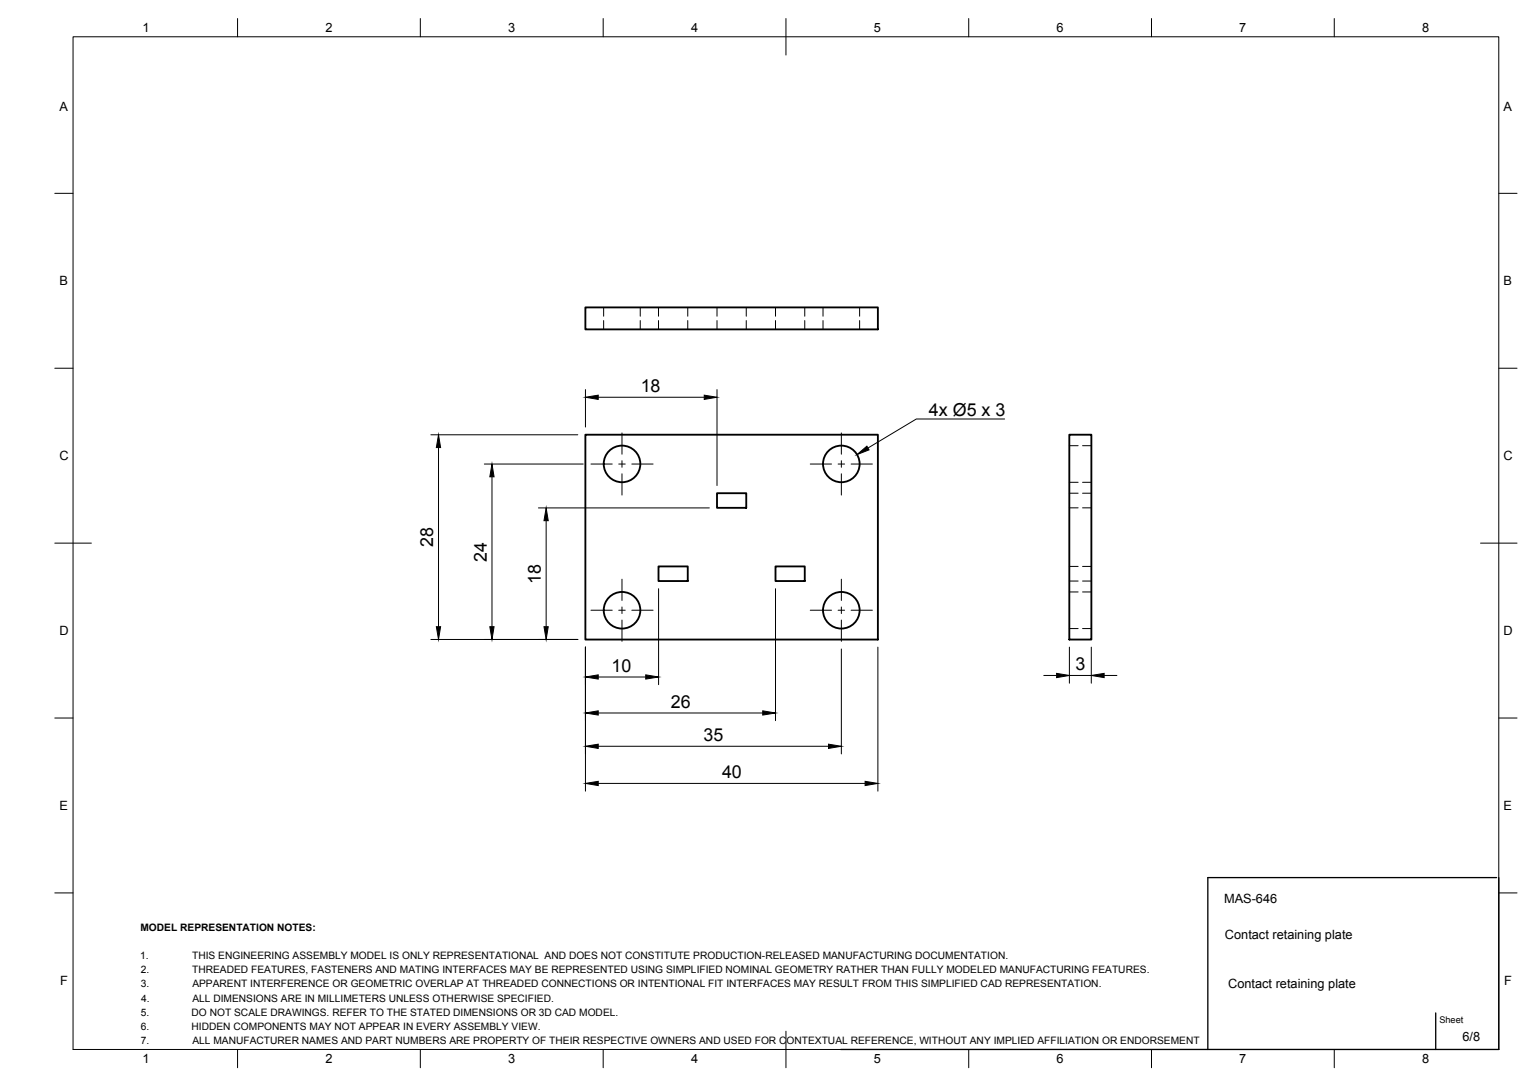
ISO-10303-21;
HEADER;
/* Generated by software containing ST-Developer
 * from STEP Tools, Inc. (www.steptools.com) 
 */

FILE_DESCRIPTION(
/* description */ ('Independent keyed three-contact power inlet for the IEC-connector des
ign category. Longer ground blade, retained contacts, wire termination
 holes and sealed bolted panel interface. Nominal custom interface; IE
C dimensional compatibility and electrical ratings are not assigned.'),

/* implementation_level */ '2;1');

FILE_NAME(
/* name */ 'Contact retaining plate.step',
/* time_stamp */ '2026-11-08T19:55:04-08:00',
/* author */ (''),
/* organization */ (''),
/* preprocessor_version */ 'ST-DEVELOPER v20.2',
/* originating_system */ 'Autodesk Translation Framework v15.17.0.0',
/* authorisation */ '');

FILE_SCHEMA (('AUTOMOTIVE_DESIGN { 1 0 10303 214 3 1 1 }'));
ENDSEC;

DATA;
#10=MECHANICAL_DESIGN_GEOMETRIC_PRESENTATION_REPRESENTATION('',(#112),#21880);
#92=SHAPE_REPRESENTATION_RELATIONSHIP('SRR','None',#21928,#102);
#102=ADVANCED_BREP_SHAPE_REPRESENTATION('',(#122),#21873);
#112=STYLED_ITEM('',(#21987),#122);
#122=MANIFOLD_SOLID_BREP('Body1',#6384);
#171=FACE_BOUND('',#918,.T.);
#172=FACE_BOUND('',#919,.T.);
#173=FACE_BOUND('',#920,.T.);
#174=FACE_BOUND('',#921,.T.);
#175=FACE_BOUND('',#922,.T.);
#176=FACE_BOUND('',#923,.T.);
#177=FACE_BOUND('',#924,.T.);
#178=FACE_BOUND('',#926,.T.);
#179=FACE_BOUND('',#927,.T.);
#180=FACE_BOUND('',#928,.T.);
#181=FACE_BOUND('',#929,.T.);
#182=FACE_BOUND('',#930,.T.);
#183=FACE_BOUND('',#931,.T.);
#184=FACE_BOUND('',#932,.T.);
#253=PLANE('',#6784);
#254=PLANE('',#6785);
#255=PLANE('',#6786);
#256=PLANE('',#6787);
#257=PLANE('',#6788);
#258=PLANE('',#6789);
#259=PLANE('',#6790);
#260=PLANE('',#6791);
#261=PLANE('',#6792);
#262=PLANE('',#6793);
#263=PLANE('',#6794);
#264=PLANE('',#6795);
#265=PLANE('',#6796);
#266=PLANE('',#6797);
#267=PLANE('',#6798);
#268=PLANE('',#6799);
#269=PLANE('',#6800);
#270=PLANE('',#6801);
#525=FACE_OUTER_BOUND('',#897,.T.);
#526=FACE_OUTER_BOUND('',#898,.T.);
#527=FACE_OUTER_BOUND('',#899,.T.);
#528=FACE_OUTER_BOUND('',#900,.T.);
#529=FACE_OUTER_BOUND('',#901,.T.);
#530=FACE_OUTER_BOUND('',#902,.T.);
#531=FACE_OUTER_BOUND('',#903,.T.);
#532=FACE_OUTER_BOUND('',#904,.T.);
#533=FACE_OUTER_BOUND('',#905,.T.);
#534=FACE_OUTER_BOUND('',#906,.T.);
#535=FACE_OUTER_BOUND('',#907,.T.);
#536=FACE_OUTER_BOUND('',#908,.T.);
#537=FACE_OUTER_BOUND('',#909,.T.);
#538=FACE_OUTER_BOUND('',#910,.T.);
#539=FACE_OUTER_BOUND('',#911,.T.);
#540=FACE_OUTER_BOUND('',#912,.T.);
#541=FACE_OUTER_BOUND('',#913,.T.);
#542=FACE_OUTER_BOUND('',#914,.T.);
#543=FACE_OUTER_BOUND('',#915,.T.);
#544=FACE_OUTER_BOUND('',#916,.T.);
#545=FACE_OUTER_BOUND('',#917,.T.);
#546=FACE_OUTER_BOUND('',#925,.T.);
#897=EDGE_LOOP('',(#5075,#5076,#5077,#5078));
#898=EDGE_LOOP('',(#5079,#5080,#5081,#5082));
#899=EDGE_LOOP('',(#5083,#5084,#5085,#5086));
#900=EDGE_LOOP('',(#5087,#5088,#5089,#5090));
#901=EDGE_LOOP('',(#5091,#5092,#5093,#5094));
#902=EDGE_LOOP('',(#5095,#5096,#5097,#5098));
#903=EDGE_LOOP('',(#5099,#5100,#5101,#5102));
#904=EDGE_LOOP('',(#5103,#5104,#5105,#5106));
#905=EDGE_LOOP('',(#5107,#5108,#5109,#5110));
#906=EDGE_LOOP('',(#5111,#5112,#5113,#5114));
#907=EDGE_LOOP('',(#5115,#5116,#5117,#5118));
#908=EDGE_LOOP('',(#5119,#5120,#5121,#5122));
#909=EDGE_LOOP('',(#5123,#5124,#5125,#5126));
#910=EDGE_LOOP('',(#5127,#5128,#5129,#5130));
#911=EDGE_LOOP('',(#5131,#5132,#5133,#5134));
#912=EDGE_LOOP('',(#5135,#5136,#5137,#5138));
#913=EDGE_LOOP('',(#5139,#5140,#5141,#5142));
#914=EDGE_LOOP('',(#5143,#5144,#5145,#5146));
#915=EDGE_LOOP('',(#5147,#5148,#5149,#5150));
#916=EDGE_LOOP('',(#5151,#5152,#5153,#5154));
#917=EDGE_LOOP('',(#5155,#5156,#5157,#5158));
#918=EDGE_LOOP('',(#5159,#5160,#5161,#5162));
#919=EDGE_LOOP('',(#5163,#5164,#5165,#5166));
#920=EDGE_LOOP('',(#5167,#5168,#5169,#5170));
#921=EDGE_LOOP('',(#5171));
#922=EDGE_LOOP('',(#5172));
#923=EDGE_LOOP('',(#5173));
#924=EDGE_LOOP('',(#5174));
#925=EDGE_LOOP('',(#5175,#5176,#5177,#5178));
#926=EDGE_LOOP('',(#5179,#5180,#5181,#5182));
#927=EDGE_LOOP('',(#5183,#5184,#5185,#5186));
#928=EDGE_LOOP('',(#5187,#5188,#5189,#5190));
#929=EDGE_LOOP('',(#5191));
#930=EDGE_LOOP('',(#5192));
#931=EDGE_LOOP('',(#5193));
#932=EDGE_LOOP('',(#5194));
#1128=CIRCLE('',#6773,2.5);
#1129=CIRCLE('',#6774,2.5);
#1130=CIRCLE('',#6776,2.5);
#1131=CIRCLE('',#6777,2.5);
#1132=CIRCLE('',#6779,2.5);
#1133=CIRCLE('',#6780,2.5);
#1134=CIRCLE('',#6782,2.5);
#1135=CIRCLE('',#6783,2.5);
#1787=LINE('',#16163,#2243);
#1788=LINE('',#16169,#2244);
#1789=LINE('',#16175,#2245);
#1790=LINE('',#16181,#2246);
#1791=LINE('',#16186,#2247);
#1792=LINE('',#16188,#2248);
#1793=LINE('',#16190,#2249);
#1794=LINE('',#16191,#2250);
#1795=LINE('',#16194,#2251);
#1796=LINE('',#16196,#2252);
#1797=LINE('',#16197,#2253);
#1798=LINE('',#16200,#2254);
#1799=LINE('',#16202,#2255);
#1800=LINE('',#16203,#2256);
#1801=LINE('',#16205,#2257);
#1802=LINE('',#16206,#2258);
#1803=LINE('',#16210,#2259);
#1804=LINE('',#16212,#2260);
#1805=LINE('',#16214,#2261);
#1806=LINE('',#16215,#2262);
#1807=LINE('',#16218,#2263);
#1808=LINE('',#16220,#2264);
#1809=LINE('',#16221,#2265);
#1810=LINE('',#16224,#2266);
#1811=LINE('',#16226,#2267);
#1812=LINE('',#16227,#2268);
#1813=LINE('',#16229,#2269);
#1814=LINE('',#16230,#2270);
#1815=LINE('',#16234,#2271);
#1816=LINE('',#16236,#2272);
#1817=LINE('',#16238,#2273);
#1818=LINE('',#16239,#2274);
#1819=LINE('',#16242,#2275);
#1820=LINE('',#16244,#2276);
#1821=LINE('',#16245,#2277);
#1822=LINE('',#16248,#2278);
#1823=LINE('',#16250,#2279);
#1824=LINE('',#16251,#2280);
#1825=LINE('',#16253,#2281);
#1826=LINE('',#16254,#2282);
#1827=LINE('',#16258,#2283);
#1828=LINE('',#16260,#2284);
#1829=LINE('',#16262,#2285);
#1830=LINE('',#16263,#2286);
#1831=LINE('',#16266,#2287);
#1832=LINE('',#16268,#2288);
#1833=LINE('',#16269,#2289);
#1834=LINE('',#16272,#2290);
#1835=LINE('',#16274,#2291);
#1836=LINE('',#16275,#2292);
#1837=LINE('',#16277,#2293);
#1838=LINE('',#16278,#2294);
#2243=VECTOR('',#7769,2.5);
#2244=VECTOR('',#7776,2.5);
#2245=VECTOR('',#7783,2.5);
#2246=VECTOR('',#7790,2.5);
#2247=VECTOR('',#7795,10.);
#2248=VECTOR('',#7796,10.);
#2249=VECTOR('',#7797,10.);
#2250=VECTOR('',#7798,10.);
#2251=VECTOR('',#7801,10.);
#2252=VECTOR('',#7802,10.);
#2253=VECTOR('',#7803,10.);
#2254=VECTOR('',#7806,10.);
#2255=VECTOR('',#7807,10.);
#2256=VECTOR('',#7808,10.);
#2257=VECTOR('',#7811,10.);
#2258=VECTOR('',#7812,10.);
#2259=VECTOR('',#7815,10.);
#2260=VECTOR('',#7816,10.);
#2261=VECTOR('',#7817,10.);
#2262=VECTOR('',#7818,10.);
#2263=VECTOR('',#7821,10.);
#2264=VECTOR('',#7822,10.);
#2265=VECTOR('',#7823,10.);
#2266=VECTOR('',#7826,10.);
#2267=VECTOR('',#7827,10.);
#2268=VECTOR('',#7828,10.);
#2269=VECTOR('',#7831,10.);
#2270=VECTOR('',#7832,10.);
#2271=VECTOR('',#7835,10.);
#2272=VECTOR('',#7836,10.);
#2273=VECTOR('',#7837,10.);
#2274=VECTOR('',#7838,10.);
#2275=VECTOR('',#7841,10.);
#2276=VECTOR('',#7842,10.);
#2277=VECTOR('',#7843,10.);
#2278=VECTOR('',#7846,10.);
#2279=VECTOR('',#7847,10.);
#2280=VECTOR('',#7848,10.);
#2281=VECTOR('',#7851,10.);
#2282=VECTOR('',#7852,10.);
#2283=VECTOR('',#7855,10.);
#2284=VECTOR('',#7856,10.);
#2285=VECTOR('',#7857,10.);
#2286=VECTOR('',#7858,10.);
#2287=VECTOR('',#7861,10.);
#2288=VECTOR('',#7862,10.);
#2289=VECTOR('',#7863,10.);
#2290=VECTOR('',#7866,10.);
#2291=VECTOR('',#7867,10.);
#2292=VECTOR('',#7868,10.);
#2293=VECTOR('',#7871,10.);
#2294=VECTOR('',#7872,10.);
#2795=VERTEX_POINT('',#16160);
#2796=VERTEX_POINT('',#16162);
#2797=VERTEX_POINT('',#16166);
#2798=VERTEX_POINT('',#16168);
#2799=VERTEX_POINT('',#16172);
#2800=VERTEX_POINT('',#16174);
#2801=VERTEX_POINT('',#16178);
#2802=VERTEX_POINT('',#16180);
#2803=VERTEX_POINT('',#16184);
#2804=VERTEX_POINT('',#16185);
#2805=VERTEX_POINT('',#16187);
#2806=VERTEX_POINT('',#16189);
#2807=VERTEX_POINT('',#16193);
#2808=VERTEX_POINT('',#16195);
#2809=VERTEX_POINT('',#16199);
#2810=VERTEX_POINT('',#16201);
#2811=VERTEX_POINT('',#16208);
#2812=VERTEX_POINT('',#16209);
#2813=VERTEX_POINT('',#16211);
#2814=VERTEX_POINT('',#16213);
#2815=VERTEX_POINT('',#16217);
#2816=VERTEX_POINT('',#16219);
#2817=VERTEX_POINT('',#16223);
#2818=VERTEX_POINT('',#16225);
#2819=VERTEX_POINT('',#16232);
#2820=VERTEX_POINT('',#16233);
#2821=VERTEX_POINT('',#16235);
#2822=VERTEX_POINT('',#16237);
#2823=VERTEX_POINT('',#16241);
#2824=VERTEX_POINT('',#16243);
#2825=VERTEX_POINT('',#16247);
#2826=VERTEX_POINT('',#16249);
#2827=VERTEX_POINT('',#16256);
#2828=VERTEX_POINT('',#16257);
#2829=VERTEX_POINT('',#16259);
#2830=VERTEX_POINT('',#16261);
#2831=VERTEX_POINT('',#16265);
#2832=VERTEX_POINT('',#16267);
#2833=VERTEX_POINT('',#16271);
#2834=VERTEX_POINT('',#16273);
#3597=EDGE_CURVE('',#2795,#2795,#1128,.T.);
#3598=EDGE_CURVE('',#2795,#2796,#1787,.T.);
#3599=EDGE_CURVE('',#2796,#2796,#1129,.T.);
#3600=EDGE_CURVE('',#2797,#2797,#1130,.T.);
#3601=EDGE_CURVE('',#2797,#2798,#1788,.T.);
#3602=EDGE_CURVE('',#2798,#2798,#1131,.T.);
#3603=EDGE_CURVE('',#2799,#2799,#1132,.T.);
#3604=EDGE_CURVE('',#2799,#2800,#1789,.T.);
#3605=EDGE_CURVE('',#2800,#2800,#1133,.T.);
#3606=EDGE_CURVE('',#2801,#2801,#1134,.T.);
#3607=EDGE_CURVE('',#2801,#2802,#1790,.T.);
#3608=EDGE_CURVE('',#2802,#2802,#1135,.T.);
#3609=EDGE_CURVE('',#2803,#2804,#1791,.T.);
#3610=EDGE_CURVE('',#2803,#2805,#1792,.T.);
#3611=EDGE_CURVE('',#2806,#2805,#1793,.T.);
#3612=EDGE_CURVE('',#2804,#2806,#1794,.T.);
#3613=EDGE_CURVE('',#2807,#2803,#1795,.T.);
#3614=EDGE_CURVE('',#2807,#2808,#1796,.T.);
#3615=EDGE_CURVE('',#2805,#2808,#1797,.T.);
#3616=EDGE_CURVE('',#2809,#2807,#1798,.T.);
#3617=EDGE_CURVE('',#2809,#2810,#1799,.T.);
#3618=EDGE_CURVE('',#2808,#2810,#1800,.T.);
#3619=EDGE_CURVE('',#2804,#2809,#1801,.T.);
#3620=EDGE_CURVE('',#2810,#2806,#1802,.T.);
#3621=EDGE_CURVE('',#2811,#2812,#1803,.T.);
#3622=EDGE_CURVE('',#2811,#2813,#1804,.T.);
#3623=EDGE_CURVE('',#2814,#2813,#1805,.T.);
#3624=EDGE_CURVE('',#2812,#2814,#1806,.T.);
#3625=EDGE_CURVE('',#2815,#2811,#1807,.T.);
#3626=EDGE_CURVE('',#2815,#2816,#1808,.T.);
#3627=EDGE_CURVE('',#2813,#2816,#1809,.T.);
#3628=EDGE_CURVE('',#2817,#2815,#1810,.T.);
#3629=EDGE_CURVE('',#2817,#2818,#1811,.T.);
#3630=EDGE_CURVE('',#2816,#2818,#1812,.T.);
#3631=EDGE_CURVE('',#2812,#2817,#1813,.T.);
#3632=EDGE_CURVE('',#2818,#2814,#1814,.T.);
#3633=EDGE_CURVE('',#2819,#2820,#1815,.T.);
#3634=EDGE_CURVE('',#2819,#2821,#1816,.T.);
#3635=EDGE_CURVE('',#2822,#2821,#1817,.T.);
#3636=EDGE_CURVE('',#2820,#2822,#1818,.T.);
#3637=EDGE_CURVE('',#2823,#2819,#1819,.T.);
#3638=EDGE_CURVE('',#2823,#2824,#1820,.T.);
#3639=EDGE_CURVE('',#2821,#2824,#1821,.T.);
#3640=EDGE_CURVE('',#2825,#2823,#1822,.T.);
#3641=EDGE_CURVE('',#2825,#2826,#1823,.T.);
#3642=EDGE_CURVE('',#2824,#2826,#1824,.T.);
#3643=EDGE_CURVE('',#2820,#2825,#1825,.T.);
#3644=EDGE_CURVE('',#2826,#2822,#1826,.T.);
#3645=EDGE_CURVE('',#2827,#2828,#1827,.T.);
#3646=EDGE_CURVE('',#2828,#2829,#1828,.T.);
#3647=EDGE_CURVE('',#2830,#2829,#1829,.T.);
#3648=EDGE_CURVE('',#2827,#2830,#1830,.T.);
#3649=EDGE_CURVE('',#2831,#2827,#1831,.T.);
#3650=EDGE_CURVE('',#2832,#2830,#1832,.T.);
#3651=EDGE_CURVE('',#2831,#2832,#1833,.T.);
#3652=EDGE_CURVE('',#2833,#2831,#1834,.T.);
#3653=EDGE_CURVE('',#2834,#2832,#1835,.T.);
#3654=EDGE_CURVE('',#2833,#2834,#1836,.T.);
#3655=EDGE_CURVE('',#2828,#2833,#1837,.T.);
#3656=EDGE_CURVE('',#2829,#2834,#1838,.T.);
#5075=ORIENTED_EDGE('',*,*,#3597,.F.);
#5076=ORIENTED_EDGE('',*,*,#3598,.T.);
#5077=ORIENTED_EDGE('',*,*,#3599,.F.);
#5078=ORIENTED_EDGE('',*,*,#3598,.F.);
#5079=ORIENTED_EDGE('',*,*,#3600,.F.);
#5080=ORIENTED_EDGE('',*,*,#3601,.T.);
#5081=ORIENTED_EDGE('',*,*,#3602,.F.);
#5082=ORIENTED_EDGE('',*,*,#3601,.F.);
#5083=ORIENTED_EDGE('',*,*,#3603,.F.);
#5084=ORIENTED_EDGE('',*,*,#3604,.T.);
#5085=ORIENTED_EDGE('',*,*,#3605,.F.);
#5086=ORIENTED_EDGE('',*,*,#3604,.F.);
#5087=ORIENTED_EDGE('',*,*,#3606,.F.);
#5088=ORIENTED_EDGE('',*,*,#3607,.T.);
#5089=ORIENTED_EDGE('',*,*,#3608,.F.);
#5090=ORIENTED_EDGE('',*,*,#3607,.F.);
#5091=ORIENTED_EDGE('',*,*,#3609,.F.);
#5092=ORIENTED_EDGE('',*,*,#3610,.T.);
#5093=ORIENTED_EDGE('',*,*,#3611,.F.);
#5094=ORIENTED_EDGE('',*,*,#3612,.F.);
#5095=ORIENTED_EDGE('',*,*,#3613,.F.);
#5096=ORIENTED_EDGE('',*,*,#3614,.T.);
#5097=ORIENTED_EDGE('',*,*,#3615,.F.);
#5098=ORIENTED_EDGE('',*,*,#3610,.F.);
#5099=ORIENTED_EDGE('',*,*,#3616,.F.);
#5100=ORIENTED_EDGE('',*,*,#3617,.T.);
#5101=ORIENTED_EDGE('',*,*,#3618,.F.);
#5102=ORIENTED_EDGE('',*,*,#3614,.F.);
#5103=ORIENTED_EDGE('',*,*,#3619,.F.);
#5104=ORIENTED_EDGE('',*,*,#3612,.T.);
#5105=ORIENTED_EDGE('',*,*,#3620,.F.);
#5106=ORIENTED_EDGE('',*,*,#3617,.F.);
#5107=ORIENTED_EDGE('',*,*,#3621,.F.);
#5108=ORIENTED_EDGE('',*,*,#3622,.T.);
#5109=ORIENTED_EDGE('',*,*,#3623,.F.);
#5110=ORIENTED_EDGE('',*,*,#3624,.F.);
#5111=ORIENTED_EDGE('',*,*,#3625,.F.);
#5112=ORIENTED_EDGE('',*,*,#3626,.T.);
#5113=ORIENTED_EDGE('',*,*,#3627,.F.);
#5114=ORIENTED_EDGE('',*,*,#3622,.F.);
#5115=ORIENTED_EDGE('',*,*,#3628,.F.);
#5116=ORIENTED_EDGE('',*,*,#3629,.T.);
#5117=ORIENTED_EDGE('',*,*,#3630,.F.);
#5118=ORIENTED_EDGE('',*,*,#3626,.F.);
#5119=ORIENTED_EDGE('',*,*,#3631,.F.);
#5120=ORIENTED_EDGE('',*,*,#3624,.T.);
#5121=ORIENTED_EDGE('',*,*,#3632,.F.);
#5122=ORIENTED_EDGE('',*,*,#3629,.F.);
#5123=ORIENTED_EDGE('',*,*,#3633,.F.);
#5124=ORIENTED_EDGE('',*,*,#3634,.T.);
#5125=ORIENTED_EDGE('',*,*,#3635,.F.);
#5126=ORIENTED_EDGE('',*,*,#3636,.F.);
#5127=ORIENTED_EDGE('',*,*,#3637,.F.);
#5128=ORIENTED_EDGE('',*,*,#3638,.T.);
#5129=ORIENTED_EDGE('',*,*,#3639,.F.);
#5130=ORIENTED_EDGE('',*,*,#3634,.F.);
#5131=ORIENTED_EDGE('',*,*,#3640,.F.);
#5132=ORIENTED_EDGE('',*,*,#3641,.T.);
#5133=ORIENTED_EDGE('',*,*,#3642,.F.);
#5134=ORIENTED_EDGE('',*,*,#3638,.F.);
#5135=ORIENTED_EDGE('',*,*,#3643,.F.);
#5136=ORIENTED_EDGE('',*,*,#3636,.T.);
#5137=ORIENTED_EDGE('',*,*,#3644,.F.);
#5138=ORIENTED_EDGE('',*,*,#3641,.F.);
#5139=ORIENTED_EDGE('',*,*,#3645,.T.);
#5140=ORIENTED_EDGE('',*,*,#3646,.T.);
#5141=ORIENTED_EDGE('',*,*,#3647,.F.);
#5142=ORIENTED_EDGE('',*,*,#3648,.F.);
#5143=ORIENTED_EDGE('',*,*,#3649,.T.);
#5144=ORIENTED_EDGE('',*,*,#3648,.T.);
#5145=ORIENTED_EDGE('',*,*,#3650,.F.);
#5146=ORIENTED_EDGE('',*,*,#3651,.F.);
#5147=ORIENTED_EDGE('',*,*,#3652,.T.);
#5148=ORIENTED_EDGE('',*,*,#3651,.T.);
#5149=ORIENTED_EDGE('',*,*,#3653,.F.);
#5150=ORIENTED_EDGE('',*,*,#3654,.F.);
#5151=ORIENTED_EDGE('',*,*,#3655,.T.);
#5152=ORIENTED_EDGE('',*,*,#3654,.T.);
#5153=ORIENTED_EDGE('',*,*,#3656,.F.);
#5154=ORIENTED_EDGE('',*,*,#3646,.F.);
#5155=ORIENTED_EDGE('',*,*,#3656,.T.);
#5156=ORIENTED_EDGE('',*,*,#3653,.T.);
#5157=ORIENTED_EDGE('',*,*,#3650,.T.);
#5158=ORIENTED_EDGE('',*,*,#3647,.T.);
#5159=ORIENTED_EDGE('',*,*,#3633,.T.);
#5160=ORIENTED_EDGE('',*,*,#3643,.T.);
#5161=ORIENTED_EDGE('',*,*,#3640,.T.);
#5162=ORIENTED_EDGE('',*,*,#3637,.T.);
#5163=ORIENTED_EDGE('',*,*,#3621,.T.);
#5164=ORIENTED_EDGE('',*,*,#3631,.T.);
#5165=ORIENTED_EDGE('',*,*,#3628,.T.);
#5166=ORIENTED_EDGE('',*,*,#3625,.T.);
#5167=ORIENTED_EDGE('',*,*,#3609,.T.);
#5168=ORIENTED_EDGE('',*,*,#3619,.T.);
#5169=ORIENTED_EDGE('',*,*,#3616,.T.);
#5170=ORIENTED_EDGE('',*,*,#3613,.T.);
#5171=ORIENTED_EDGE('',*,*,#3606,.T.);
#5172=ORIENTED_EDGE('',*,*,#3603,.T.);
#5173=ORIENTED_EDGE('',*,*,#3600,.T.);
#5174=ORIENTED_EDGE('',*,*,#3597,.T.);
#5175=ORIENTED_EDGE('',*,*,#3655,.F.);
#5176=ORIENTED_EDGE('',*,*,#3645,.F.);
#5177=ORIENTED_EDGE('',*,*,#3649,.F.);
#5178=ORIENTED_EDGE('',*,*,#3652,.F.);
#5179=ORIENTED_EDGE('',*,*,#3635,.T.);
#5180=ORIENTED_EDGE('',*,*,#3639,.T.);
#5181=ORIENTED_EDGE('',*,*,#3642,.T.);
#5182=ORIENTED_EDGE('',*,*,#3644,.T.);
#5183=ORIENTED_EDGE('',*,*,#3623,.T.);
#5184=ORIENTED_EDGE('',*,*,#3627,.T.);
#5185=ORIENTED_EDGE('',*,*,#3630,.T.);
#5186=ORIENTED_EDGE('',*,*,#3632,.T.);
#5187=ORIENTED_EDGE('',*,*,#3611,.T.);
#5188=ORIENTED_EDGE('',*,*,#3615,.T.);
#5189=ORIENTED_EDGE('',*,*,#3618,.T.);
#5190=ORIENTED_EDGE('',*,*,#3620,.T.);
#5191=ORIENTED_EDGE('',*,*,#3608,.T.);
#5192=ORIENTED_EDGE('',*,*,#3605,.T.);
#5193=ORIENTED_EDGE('',*,*,#3602,.T.);
#5194=ORIENTED_EDGE('',*,*,#3599,.T.);
#5959=CYLINDRICAL_SURFACE('',#6772,2.5);
#5960=CYLINDRICAL_SURFACE('',#6775,2.5);
#5961=CYLINDRICAL_SURFACE('',#6778,2.5);
#5962=CYLINDRICAL_SURFACE('',#6781,2.5);
#6237=ADVANCED_FACE('',(#525),#5959,.F.);
#6238=ADVANCED_FACE('',(#526),#5960,.F.);
#6239=ADVANCED_FACE('',(#527),#5961,.F.);
#6240=ADVANCED_FACE('',(#528),#5962,.F.);
#6241=ADVANCED_FACE('',(#529),#253,.F.);
#6242=ADVANCED_FACE('',(#530),#254,.F.);
#6243=ADVANCED_FACE('',(#531),#255,.F.);
#6244=ADVANCED_FACE('',(#532),#256,.F.);
#6245=ADVANCED_FACE('',(#533),#257,.F.);
#6246=ADVANCED_FACE('',(#534),#258,.F.);
#6247=ADVANCED_FACE('',(#535),#259,.F.);
#6248=ADVANCED_FACE('',(#536),#260,.F.);
#6249=ADVANCED_FACE('',(#537),#261,.F.);
#6250=ADVANCED_FACE('',(#538),#262,.F.);
#6251=ADVANCED_FACE('',(#539),#263,.F.);
#6252=ADVANCED_FACE('',(#540),#264,.F.);
#6253=ADVANCED_FACE('',(#541),#265,.T.);
#6254=ADVANCED_FACE('',(#542),#266,.T.);
#6255=ADVANCED_FACE('',(#543),#267,.T.);
#6256=ADVANCED_FACE('',(#544),#268,.T.);
#6257=ADVANCED_FACE('',(#545,#171,#172,#173,#174,#175,#176,#177),#269,.T.);
#6258=ADVANCED_FACE('',(#546,#178,#179,#180,#181,#182,#183,#184),#270,.F.);
#6384=CLOSED_SHELL('',(#6237,#6238,#6239,#6240,#6241,#6242,#6243,#6244,
#6245,#6246,#6247,#6248,#6249,#6250,#6251,#6252,#6253,#6254,#6255,#6256,
#6257,#6258));
#6771=AXIS2_PLACEMENT_3D('',#16158,#7763,#7764);
#6772=AXIS2_PLACEMENT_3D('',#16159,#7765,#7766);
#6773=AXIS2_PLACEMENT_3D('',#16161,#7767,#7768);
#6774=AXIS2_PLACEMENT_3D('',#16164,#7770,#7771);
#6775=AXIS2_PLACEMENT_3D('',#16165,#7772,#7773);
#6776=AXIS2_PLACEMENT_3D('',#16167,#7774,#7775);
#6777=AXIS2_PLACEMENT_3D('',#16170,#7777,#7778);
#6778=AXIS2_PLACEMENT_3D('',#16171,#7779,#7780);
#6779=AXIS2_PLACEMENT_3D('',#16173,#7781,#7782);
#6780=AXIS2_PLACEMENT_3D('',#16176,#7784,#7785);
#6781=AXIS2_PLACEMENT_3D('',#16177,#7786,#7787);
#6782=AXIS2_PLACEMENT_3D('',#16179,#7788,#7789);
#6783=AXIS2_PLACEMENT_3D('',#16182,#7791,#7792);
#6784=AXIS2_PLACEMENT_3D('',#16183,#7793,#7794);
#6785=AXIS2_PLACEMENT_3D('',#16192,#7799,#7800);
#6786=AXIS2_PLACEMENT_3D('',#16198,#7804,#7805);
#6787=AXIS2_PLACEMENT_3D('',#16204,#7809,#7810);
#6788=AXIS2_PLACEMENT_3D('',#16207,#7813,#7814);
#6789=AXIS2_PLACEMENT_3D('',#16216,#7819,#7820);
#6790=AXIS2_PLACEMENT_3D('',#16222,#7824,#7825);
#6791=AXIS2_PLACEMENT_3D('',#16228,#7829,#7830);
#6792=AXIS2_PLACEMENT_3D('',#16231,#7833,#7834);
#6793=AXIS2_PLACEMENT_3D('',#16240,#7839,#7840);
#6794=AXIS2_PLACEMENT_3D('',#16246,#7844,#7845);
#6795=AXIS2_PLACEMENT_3D('',#16252,#7849,#7850);
#6796=AXIS2_PLACEMENT_3D('',#16255,#7853,#7854);
#6797=AXIS2_PLACEMENT_3D('',#16264,#7859,#7860);
#6798=AXIS2_PLACEMENT_3D('',#16270,#7864,#7865);
#6799=AXIS2_PLACEMENT_3D('',#16276,#7869,#7870);
#6800=AXIS2_PLACEMENT_3D('',#16279,#7873,#7874);
#6801=AXIS2_PLACEMENT_3D('',#16280,#7875,#7876);
#7763=DIRECTION('axis',(0.,0.,1.));
#7764=DIRECTION('refdir',(1.,0.,0.));
#7765=DIRECTION('center_axis',(0.,0.,-1.));
#7766=DIRECTION('ref_axis',(1.,0.,0.));
#7767=DIRECTION('center_axis',(0.,0.,-1.));
#7768=DIRECTION('ref_axis',(1.,0.,0.));
#7769=DIRECTION('',(0.,0.,-1.));
#7770=DIRECTION('center_axis',(0.,0.,1.));
#7771=DIRECTION('ref_axis',(1.,0.,0.));
#7772=DIRECTION('center_axis',(0.,0.,-1.));
#7773=DIRECTION('ref_axis',(1.,0.,0.));
#7774=DIRECTION('center_axis',(0.,0.,-1.));
#7775=DIRECTION('ref_axis',(1.,0.,0.));
#7776=DIRECTION('',(0.,0.,-1.));
#7777=DIRECTION('center_axis',(0.,0.,1.));
#7778=DIRECTION('ref_axis',(1.,0.,0.));
#7779=DIRECTION('center_axis',(0.,0.,-1.));
#7780=DIRECTION('ref_axis',(1.,0.,0.));
#7781=DIRECTION('center_axis',(0.,0.,-1.));
#7782=DIRECTION('ref_axis',(1.,0.,0.));
#7783=DIRECTION('',(0.,0.,-1.));
#7784=DIRECTION('center_axis',(0.,0.,1.));
#7785=DIRECTION('ref_axis',(1.,0.,0.));
#7786=DIRECTION('center_axis',(0.,0.,-1.));
#7787=DIRECTION('ref_axis',(1.,0.,0.));
#7788=DIRECTION('center_axis',(0.,0.,-1.));
#7789=DIRECTION('ref_axis',(1.,0.,0.));
#7790=DIRECTION('',(0.,0.,-1.));
#7791=DIRECTION('center_axis',(0.,0.,1.));
#7792=DIRECTION('ref_axis',(1.,0.,0.));
#7793=DIRECTION('center_axis',(0.,-1.,0.));
#7794=DIRECTION('ref_axis',(-1.,0.,0.));
#7795=DIRECTION('',(-1.,0.,0.));
#7796=DIRECTION('',(0.,0.,-1.));
#7797=DIRECTION('',(1.,0.,0.));
#7798=DIRECTION('',(0.,0.,-1.));
#7799=DIRECTION('center_axis',(1.,0.,0.));
#7800=DIRECTION('ref_axis',(0.,-1.,0.));
#7801=DIRECTION('',(0.,-1.,0.));
#7802=DIRECTION('',(0.,0.,-1.));
#7803=DIRECTION('',(0.,1.,0.));
#7804=DIRECTION('center_axis',(0.,1.,0.));
#7805=DIRECTION('ref_axis',(1.,0.,0.));
#7806=DIRECTION('',(1.,0.,0.));
#7807=DIRECTION('',(0.,0.,-1.));
#7808=DIRECTION('',(-1.,0.,0.));
#7809=DIRECTION('center_axis',(-1.,0.,0.));
#7810=DIRECTION('ref_axis',(0.,1.,0.));
#7811=DIRECTION('',(0.,1.,0.));
#7812=DIRECTION('',(0.,-1.,0.));
#7813=DIRECTION('center_axis',(0.,-1.,0.));
#7814=DIRECTION('ref_axis',(-1.,0.,0.));
#7815=DIRECTION('',(-1.,0.,0.));
#7816=DIRECTION('',(0.,0.,-1.));
#7817=DIRECTION('',(1.,0.,0.));
#7818=DIRECTION('',(0.,0.,-1.));
#7819=DIRECTION('center_axis',(1.,0.,0.));
#7820=DIRECTION('ref_axis',(0.,-1.,0.));
#7821=DIRECTION('',(0.,-1.,0.));
#7822=DIRECTION('',(0.,0.,-1.));
#7823=DIRECTION('',(0.,1.,0.));
#7824=DIRECTION('center_axis',(0.,1.,0.));
#7825=DIRECTION('ref_axis',(1.,0.,0.));
#7826=DIRECTION('',(1.,0.,0.));
#7827=DIRECTION('',(0.,0.,-1.));
#7828=DIRECTION('',(-1.,0.,0.));
#7829=DIRECTION('center_axis',(-1.,0.,0.));
#7830=DIRECTION('ref_axis',(0.,1.,0.));
#7831=DIRECTION('',(0.,1.,0.));
#7832=DIRECTION('',(0.,-1.,0.));
#7833=DIRECTION('center_axis',(0.,-1.,0.));
#7834=DIRECTION('ref_axis',(-1.,0.,0.));
#7835=DIRECTION('',(-1.,0.,0.));
#7836=DIRECTION('',(0.,0.,-1.));
#7837=DIRECTION('',(1.,0.,0.));
#7838=DIRECTION('',(0.,0.,-1.));
#7839=DIRECTION('center_axis',(1.,0.,0.));
#7840=DIRECTION('ref_axis',(0.,-1.,0.));
#7841=DIRECTION('',(0.,-1.,0.));
#7842=DIRECTION('',(0.,0.,-1.));
#7843=DIRECTION('',(0.,1.,0.));
#7844=DIRECTION('center_axis',(0.,1.,0.));
#7845=DIRECTION('ref_axis',(1.,0.,0.));
#7846=DIRECTION('',(1.,0.,0.));
#7847=DIRECTION('',(0.,0.,-1.));
#7848=DIRECTION('',(-1.,0.,0.));
#7849=DIRECTION('center_axis',(-1.,0.,0.));
#7850=DIRECTION('ref_axis',(0.,1.,0.));
#7851=DIRECTION('',(0.,1.,0.));
#7852=DIRECTION('',(0.,-1.,0.));
#7853=DIRECTION('center_axis',(0.,1.,0.));
#7854=DIRECTION('ref_axis',(-1.,0.,0.));
#7855=DIRECTION('',(-1.,0.,0.));
#7856=DIRECTION('',(0.,0.,1.));
#7857=DIRECTION('',(-1.,0.,0.));
#7858=DIRECTION('',(0.,0.,1.));
#7859=DIRECTION('center_axis',(1.,0.,0.));
#7860=DIRECTION('ref_axis',(0.,1.,0.));
#7861=DIRECTION('',(0.,1.,0.));
#7862=DIRECTION('',(0.,1.,0.));
#7863=DIRECTION('',(0.,0.,1.));
#7864=DIRECTION('center_axis',(0.,-1.,0.));
#7865=DIRECTION('ref_axis',(1.,0.,0.));
#7866=DIRECTION('',(1.,0.,0.));
#7867=DIRECTION('',(1.,0.,0.));
#7868=DIRECTION('',(0.,0.,1.));
#7869=DIRECTION('center_axis',(-1.,0.,0.));
#7870=DIRECTION('ref_axis',(0.,-1.,0.));
#7871=DIRECTION('',(0.,-1.,0.));
#7872=DIRECTION('',(0.,-1.,0.));
#7873=DIRECTION('center_axis',(0.,0.,1.));
#7874=DIRECTION('ref_axis',(1.,0.,0.));
#7875=DIRECTION('center_axis',(0.,0.,1.));
#7876=DIRECTION('ref_axis',(1.,0.,0.));
#16158=CARTESIAN_POINT('',(0.,0.,0.));
#16159=CARTESIAN_POINT('Origin',(15.,-10.,1.5));
#16160=CARTESIAN_POINT('',(12.5,-10.,3.));
#16161=CARTESIAN_POINT('Origin',(15.,-10.,3.));
#16162=CARTESIAN_POINT('',(12.5,-10.,0.));
#16163=CARTESIAN_POINT('',(12.5,-10.,1.5));
#16164=CARTESIAN_POINT('Origin',(15.,-10.,0.));
#16165=CARTESIAN_POINT('Origin',(-15.,-10.,1.5));
#16166=CARTESIAN_POINT('',(-17.5,-10.,3.));
#16167=CARTESIAN_POINT('Origin',(-15.,-10.,3.));
#16168=CARTESIAN_POINT('',(-17.5,-10.,0.));
#16169=CARTESIAN_POINT('',(-17.5,-10.,1.5));
#16170=CARTESIAN_POINT('Origin',(-15.,-10.,0.));
#16171=CARTESIAN_POINT('Origin',(-15.,10.,1.5));
#16172=CARTESIAN_POINT('',(-17.5,10.,3.));
#16173=CARTESIAN_POINT('Origin',(-15.,10.,3.));
#16174=CARTESIAN_POINT('',(-17.5,10.,0.));
#16175=CARTESIAN_POINT('',(-17.5,10.,1.5));
#16176=CARTESIAN_POINT('Origin',(-15.,10.,0.));
#16177=CARTESIAN_POINT('Origin',(15.,10.,1.5));
#16178=CARTESIAN_POINT('',(12.5,10.,3.));
#16179=CARTESIAN_POINT('Origin',(15.,10.,3.));
#16180=CARTESIAN_POINT('',(12.5,10.,0.));
#16181=CARTESIAN_POINT('',(12.5,10.,1.5));
#16182=CARTESIAN_POINT('Origin',(15.,10.,0.));
#16183=CARTESIAN_POINT('Origin',(-6.,-6.,3.));
#16184=CARTESIAN_POINT('',(-6.,-6.,3.));
#16185=CARTESIAN_POINT('',(-10.,-6.,3.));
#16186=CARTESIAN_POINT('',(-3.,-6.,3.));
#16187=CARTESIAN_POINT('',(-6.,-6.,0.));
#16188=CARTESIAN_POINT('',(-6.,-6.,3.));
#16189=CARTESIAN_POINT('',(-10.,-6.,0.));
#16190=CARTESIAN_POINT('',(-3.,-6.,0.));
#16191=CARTESIAN_POINT('',(-10.,-6.,3.));
#16192=CARTESIAN_POINT('Origin',(-6.,-4.,3.));
#16193=CARTESIAN_POINT('',(-6.,-4.,3.));
#16194=CARTESIAN_POINT('',(-6.,-2.,3.));
#16195=CARTESIAN_POINT('',(-6.,-4.,0.));
#16196=CARTESIAN_POINT('',(-6.,-4.,3.));
#16197=CARTESIAN_POINT('',(-6.,-2.,0.));
#16198=CARTESIAN_POINT('Origin',(-10.,-4.,3.));
#16199=CARTESIAN_POINT('',(-10.,-4.,3.));
#16200=CARTESIAN_POINT('',(-5.,-4.,3.));
#16201=CARTESIAN_POINT('',(-10.,-4.,0.));
#16202=CARTESIAN_POINT('',(-10.,-4.,3.));
#16203=CARTESIAN_POINT('',(-5.,-4.,0.));
#16204=CARTESIAN_POINT('Origin',(-10.,-6.,3.));
#16205=CARTESIAN_POINT('',(-10.,-3.,3.));
#16206=CARTESIAN_POINT('',(-10.,-3.,0.));
#16207=CARTESIAN_POINT('Origin',(10.,-6.,3.));
#16208=CARTESIAN_POINT('',(10.,-6.,3.));
#16209=CARTESIAN_POINT('',(6.,-6.,3.));
#16210=CARTESIAN_POINT('',(5.,-6.,3.));
#16211=CARTESIAN_POINT('',(10.,-6.,0.));
#16212=CARTESIAN_POINT('',(10.,-6.,3.));
#16213=CARTESIAN_POINT('',(6.,-6.,0.));
#16214=CARTESIAN_POINT('',(5.,-6.,0.));
#16215=CARTESIAN_POINT('',(6.,-6.,3.));
#16216=CARTESIAN_POINT('Origin',(10.,-4.,3.));
#16217=CARTESIAN_POINT('',(10.,-4.,3.));
#16218=CARTESIAN_POINT('',(10.,-2.,3.));
#16219=CARTESIAN_POINT('',(10.,-4.,0.));
#16220=CARTESIAN_POINT('',(10.,-4.,3.));
#16221=CARTESIAN_POINT('',(10.,-2.,0.));
#16222=CARTESIAN_POINT('Origin',(6.,-4.,3.));
#16223=CARTESIAN_POINT('',(6.,-4.,3.));
#16224=CARTESIAN_POINT('',(3.,-4.,3.));
#16225=CARTESIAN_POINT('',(6.,-4.,0.));
#16226=CARTESIAN_POINT('',(6.,-4.,3.));
#16227=CARTESIAN_POINT('',(3.,-4.,0.));
#16228=CARTESIAN_POINT('Origin',(6.,-6.,3.));
#16229=CARTESIAN_POINT('',(6.,-3.,3.));
#16230=CARTESIAN_POINT('',(6.,-3.,0.));
#16231=CARTESIAN_POINT('Origin',(2.,4.,3.));
#16232=CARTESIAN_POINT('',(2.,4.,3.));
#16233=CARTESIAN_POINT('',(-2.,4.,3.));
#16234=CARTESIAN_POINT('',(1.,4.,3.));
#16235=CARTESIAN_POINT('',(2.,4.,0.));
#16236=CARTESIAN_POINT('',(2.,4.,3.));
#16237=CARTESIAN_POINT('',(-2.,4.,0.));
#16238=CARTESIAN_POINT('',(1.,4.,0.));
#16239=CARTESIAN_POINT('',(-2.,4.,3.));
#16240=CARTESIAN_POINT('Origin',(2.,6.,3.));
#16241=CARTESIAN_POINT('',(2.,6.,3.));
#16242=CARTESIAN_POINT('',(2.,3.,3.));
#16243=CARTESIAN_POINT('',(2.,6.,0.));
#16244=CARTESIAN_POINT('',(2.,6.,3.));
#16245=CARTESIAN_POINT('',(2.,3.,0.));
#16246=CARTESIAN_POINT('Origin',(-2.,6.,3.));
#16247=CARTESIAN_POINT('',(-2.,6.,3.));
#16248=CARTESIAN_POINT('',(-1.,6.,3.));
#16249=CARTESIAN_POINT('',(-2.,6.,0.));
#16250=CARTESIAN_POINT('',(-2.,6.,3.));
#16251=CARTESIAN_POINT('',(-1.,6.,0.));
#16252=CARTESIAN_POINT('Origin',(-2.,4.,3.));
#16253=CARTESIAN_POINT('',(-2.,2.,3.));
#16254=CARTESIAN_POINT('',(-2.,2.,0.));
#16255=CARTESIAN_POINT('Origin',(20.,14.,0.));
#16256=CARTESIAN_POINT('',(20.,14.,0.));
#16257=CARTESIAN_POINT('',(-20.,14.,0.));
#16258=CARTESIAN_POINT('',(20.,14.,0.));
#16259=CARTESIAN_POINT('',(-20.,14.,3.));
#16260=CARTESIAN_POINT('',(-20.,14.,0.));
#16261=CARTESIAN_POINT('',(20.,14.,3.));
#16262=CARTESIAN_POINT('',(20.,14.,3.));
#16263=CARTESIAN_POINT('',(20.,14.,0.));
#16264=CARTESIAN_POINT('Origin',(20.,-14.,0.));
#16265=CARTESIAN_POINT('',(20.,-14.,0.));
#16266=CARTESIAN_POINT('',(20.,-14.,0.));
#16267=CARTESIAN_POINT('',(20.,-14.,3.));
#16268=CARTESIAN_POINT('',(20.,-14.,3.));
#16269=CARTESIAN_POINT('',(20.,-14.,0.));
#16270=CARTESIAN_POINT('Origin',(-20.,-14.,0.));
#16271=CARTESIAN_POINT('',(-20.,-14.,0.));
#16272=CARTESIAN_POINT('',(-20.,-14.,0.));
#16273=CARTESIAN_POINT('',(-20.,-14.,3.));
#16274=CARTESIAN_POINT('',(-20.,-14.,3.));
#16275=CARTESIAN_POINT('',(-20.,-14.,0.));
#16276=CARTESIAN_POINT('Origin',(-20.,14.,0.));
#16277=CARTESIAN_POINT('',(-20.,14.,0.));
#16278=CARTESIAN_POINT('',(-20.,14.,3.));
#16279=CARTESIAN_POINT('Origin',(0.,0.,3.));
#16280=CARTESIAN_POINT('Origin',(0.,0.,0.));
#21861=UNCERTAINTY_MEASURE_WITH_UNIT(LENGTH_MEASURE(0.01),#21881,
'DISTANCE_ACCURACY_VALUE',
'Maximum model space distance between geometric entities at asserted c
onnectivities');
#21868=UNCERTAINTY_MEASURE_WITH_UNIT(LENGTH_MEASURE(0.01),#21881,
'DISTANCE_ACCURACY_VALUE',
'Maximum model space distance between geometric entities at asserted c
onnectivities');
#21873=(
GEOMETRIC_REPRESENTATION_CONTEXT(3)
GLOBAL_UNCERTAINTY_ASSIGNED_CONTEXT((#21861))
GLOBAL_UNIT_ASSIGNED_CONTEXT((#21881,#21883,#21884))
REPRESENTATION_CONTEXT('','3D')
);
#21880=(
GEOMETRIC_REPRESENTATION_CONTEXT(3)
GLOBAL_UNCERTAINTY_ASSIGNED_CONTEXT((#21868))
GLOBAL_UNIT_ASSIGNED_CONTEXT((#21881,#21883,#21884))
REPRESENTATION_CONTEXT('','3D')
);
#21881=(
LENGTH_UNIT()
NAMED_UNIT(*)
SI_UNIT(.MILLI.,.METRE.)
);
#21883=(
NAMED_UNIT(*)
PLANE_ANGLE_UNIT()
SI_UNIT($,.RADIAN.)
);
#21884=(
NAMED_UNIT(*)
SI_UNIT($,.STERADIAN.)
SOLID_ANGLE_UNIT()
);
#21889=SHAPE_DEFINITION_REPRESENTATION(#21900,#21928);
#21900=PRODUCT_DEFINITION_SHAPE('',$,#21940);
#21928=SHAPE_REPRESENTATION('',(#6771),#21873);
#21935=PRODUCT_DEFINITION_CONTEXT('part definition',#21970,'design');
#21940=PRODUCT_DEFINITION('Contact retaining plate',
'Contact retaining plate',#21951,#21935);
#21951=PRODUCT_DEFINITION_FORMATION('',$,#21976);
#21970=APPLICATION_CONTEXT(
'Core Data for Automotive Mechanical Design Process');
#21971=PRODUCT_CONTEXT('part definition',#21970,'mechanical');
#21976=PRODUCT('Contact retaining plate','Contact retaining plate',$,(#21971));
#21987=PRESENTATION_STYLE_ASSIGNMENT((#21993));
#21993=SURFACE_STYLE_USAGE(.BOTH.,#21999);
#21999=SURFACE_SIDE_STYLE('',(#22005));
#22005=SURFACE_STYLE_FILL_AREA(#22011);
#22011=FILL_AREA_STYLE('Sky blue',(#22017));
#22017=FILL_AREA_STYLE_COLOUR('Sky blue',#22023);
#22023=COLOUR_RGB('Sky blue',0.317647058823529,0.686274509803922,0.890196078431372);
ENDSEC;
END-ISO-10303-21;
